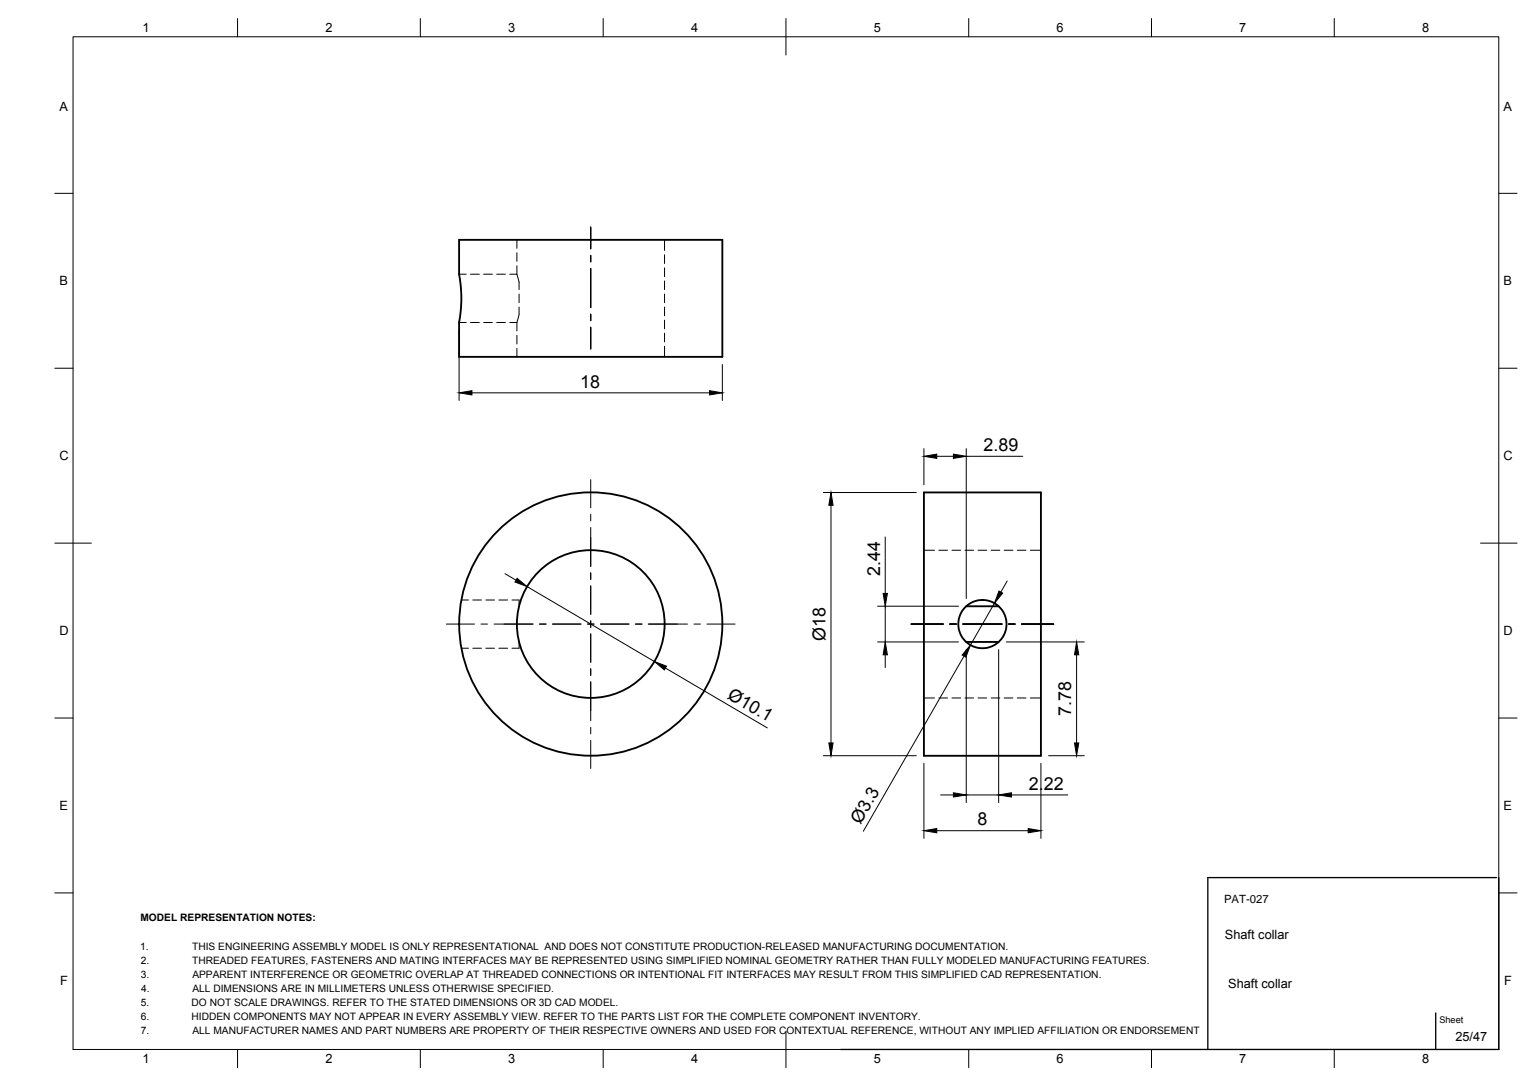
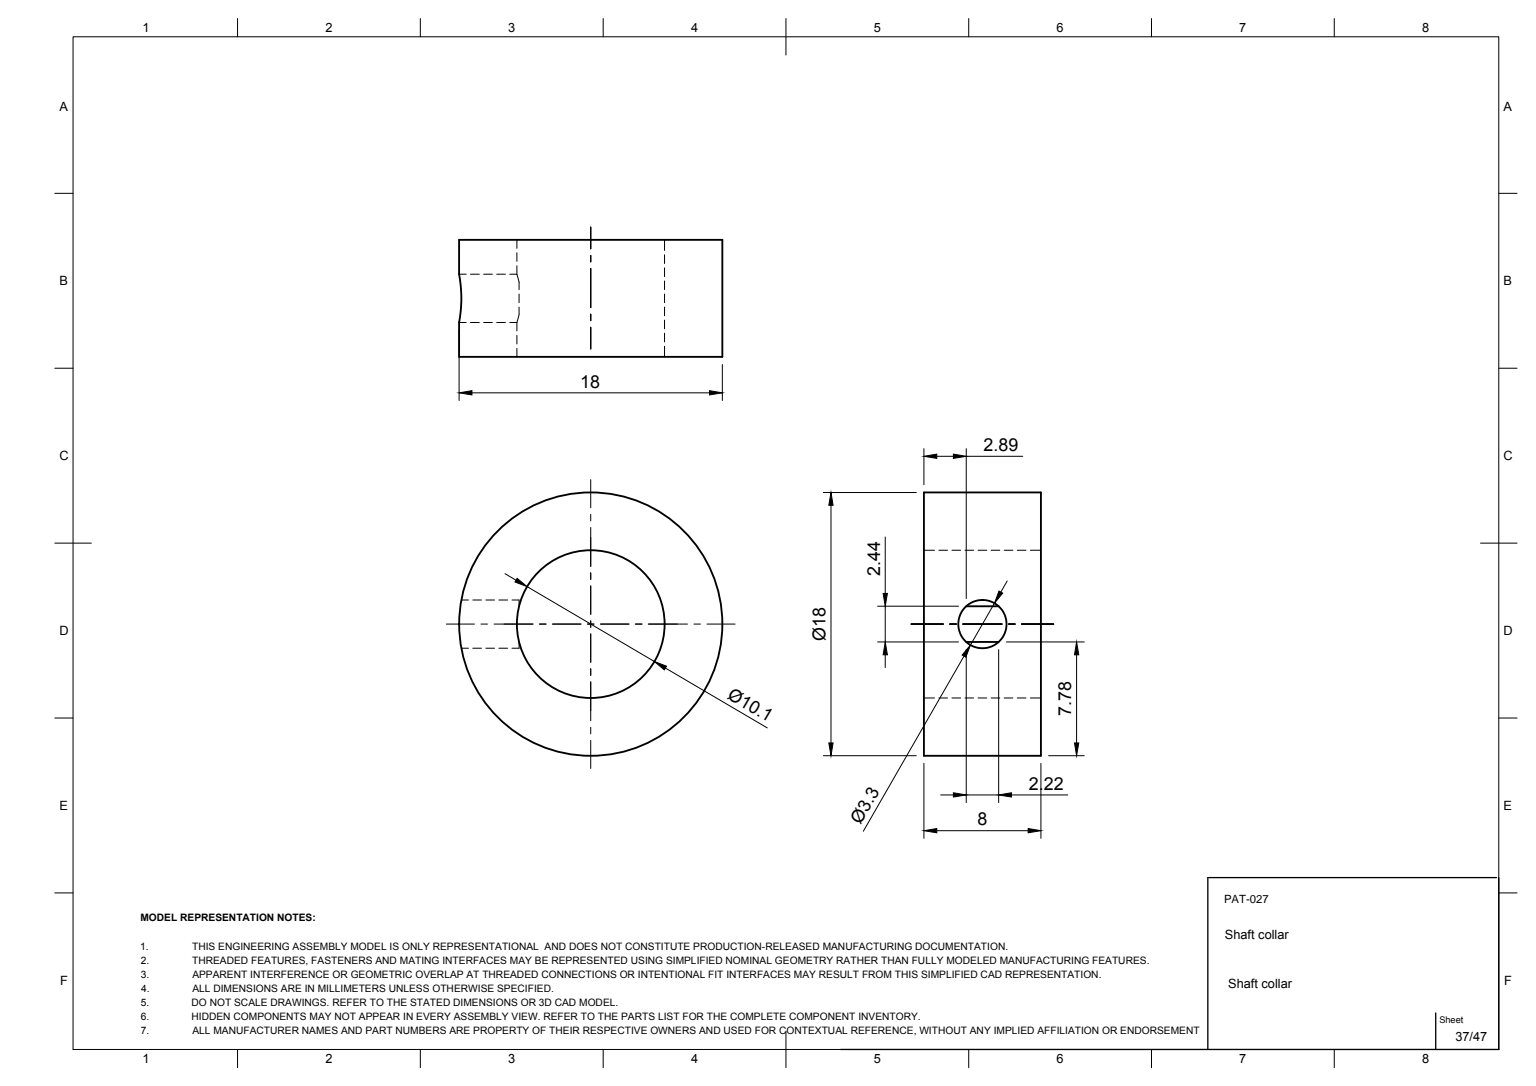
ISO-10303-21;
HEADER;
/* Generated by software containing ST-Developer
 * from STEP Tools, Inc. (www.steptools.com) 
 */

FILE_DESCRIPTION(
/* description */ ('Crank-driven oscillating fan base (mechanism only)'),

/* implementation_level */ '2;1');

FILE_NAME(
/* name */ 'Shaft collar.step',
/* time_stamp */ '2026-10-28T03:25:00-07:00',
/* author */ (''),
/* organization */ (''),
/* preprocessor_version */ 'ST-DEVELOPER v20.2',
/* originating_system */ 'Autodesk Translation Framework v15.17.0.0',
/* authorisation */ '');

FILE_SCHEMA (('AUTOMOTIVE_DESIGN { 1 0 10303 214 3 1 1 }'));
ENDSEC;

DATA;
#10=MECHANICAL_DESIGN_GEOMETRIC_PRESENTATION_REPRESENTATION('',(#462),#11916);
#342=B_SPLINE_CURVE_WITH_KNOTS('',3,(#10852,#10853,#10854,#10855,#10856,
#10857,#10858,#10859,#10860,#10861,#10862,#10863,#10864,#10865),
 .UNSPECIFIED.,.F.,.F.,(4,2,2,2,2,2,4),(0.618551524396293,0.626563103102765,
0.689203386094988,0.751843669087211,0.814483952079434,0.877124235071657,
0.88513581377813),.UNSPECIFIED.);
#343=B_SPLINE_CURVE_WITH_KNOTS('',3,(#10869,#10870,#10871,#10872,#10873,
#10874,#10875,#10876),.UNSPECIFIED.,.F.,.F.,(4,2,2,4),(0.250614556362404,
0.313254839354627,0.37589512234685,0.383906701053323),.UNSPECIFIED.);
#344=B_SPLINE_CURVE_WITH_KNOTS('',3,(#10880,#10881,#10882,#10883,#10884,
#10885,#10886,#10887,#10888,#10889,#10890,#10891,#10892,#10893,#10894,#10895,
#10896,#10897,#10898,#10899,#10900,#10901,#10902,#10903,#10904,#10905),
 .UNSPECIFIED.,.F.,.F.,(4,2,2,2,2,2,2,2,2,2,2,2,4),(0.,0.0623062782223143,
0.124612556444629,0.186916384615149,0.249220212785669,0.31152404095619,
0.37382786912671,0.436134147349024,0.498440425571339,0.560746703793653,
0.623052982015967,0.685356810186488,0.747660638357008),.UNSPECIFIED.);
#345=B_SPLINE_CURVE_WITH_KNOTS('',3,(#10906,#10907,#10908,#10909,#10910,
#10911,#10912,#10913,#10914,#10915),.UNSPECIFIED.,.F.,.F.,(4,2,2,2,4),(0.747660638357008,
0.809964466527528,0.872268294698049,0.934574572920363,0.996880851142677),
 .UNSPECIFIED.);
#346=B_SPLINE_CURVE_WITH_KNOTS('',3,(#10916,#10917,#10918,#10919,#10920,
#10921,#10922,#10923),.UNSPECIFIED.,.F.,.F.,(4,2,2,4),(0.117322411671485,
0.125333990377958,0.187974273370181,0.250614556362404),.UNSPECIFIED.);
#374=SHAPE_REPRESENTATION_RELATIONSHIP('SRR','None',#12100,#414);
#414=ADVANCED_BREP_SHAPE_REPRESENTATION('',(#509),#11891);
#462=STYLED_ITEM('',(#12375),#509);
#509=MANIFOLD_SOLID_BREP('Body1',#6093);
#626=FACE_BOUND('',#1559,.T.);
#627=FACE_BOUND('',#1561,.T.);
#628=FACE_BOUND('',#1563,.T.);
#629=FACE_BOUND('',#1565,.T.);
#782=PLANE('',#7013);
#783=PLANE('',#7017);
#784=PLANE('',#7024);
#785=PLANE('',#7025);
#1084=FACE_OUTER_BOUND('',#1555,.T.);
#1085=FACE_OUTER_BOUND('',#1556,.T.);
#1086=FACE_OUTER_BOUND('',#1557,.T.);
#1087=FACE_OUTER_BOUND('',#1558,.T.);
#1088=FACE_OUTER_BOUND('',#1560,.T.);
#1089=FACE_OUTER_BOUND('',#1562,.T.);
#1090=FACE_OUTER_BOUND('',#1564,.T.);
#1555=EDGE_LOOP('',(#4894,#4895));
#1556=EDGE_LOOP('',(#4896,#4897,#4898,#4899,#4900,#4901,#4902,#4903,#4904));
#1557=EDGE_LOOP('',(#4905,#4906));
#1558=EDGE_LOOP('',(#4907,#4908,#4909,#4910));
#1559=EDGE_LOOP('',(#4911,#4912,#4913,#4914,#4915));
#1560=EDGE_LOOP('',(#4916,#4917,#4918,#4919));
#1561=EDGE_LOOP('',(#4920,#4921));
#1562=EDGE_LOOP('',(#4922));
#1563=EDGE_LOOP('',(#4923));
#1564=EDGE_LOOP('',(#4924));
#1565=EDGE_LOOP('',(#4925));
#1956=LINE('',#10848,#2289);
#1957=LINE('',#10878,#2290);
#1958=LINE('',#10925,#2291);
#1959=LINE('',#10930,#2292);
#1960=LINE('',#10936,#2293);
#2289=VECTOR('',#8479,1.);
#2290=VECTOR('',#8486,0.165);
#2291=VECTOR('',#8489,1.);
#2292=VECTOR('',#8494,0.505);
#2293=VECTOR('',#8501,0.9);
#2693=CIRCLE('',#7014,0.165);
#2694=CIRCLE('',#7016,0.165);
#2695=CIRCLE('',#7019,0.505);
#2696=CIRCLE('',#7020,0.505);
#2697=CIRCLE('',#7022,0.9);
#2698=CIRCLE('',#7023,0.9);
#3114=VERTEX_POINT('',#10846);
#3115=VERTEX_POINT('',#10847);
#3116=VERTEX_POINT('',#10851);
#3117=VERTEX_POINT('',#10866);
#3118=VERTEX_POINT('',#10868);
#3119=VERTEX_POINT('',#10877);
#3120=VERTEX_POINT('',#10879);
#3121=VERTEX_POINT('',#10927);
#3122=VERTEX_POINT('',#10929);
#3123=VERTEX_POINT('',#10933);
#3124=VERTEX_POINT('',#10935);
#3742=EDGE_CURVE('',#3114,#3115,#1956,.T.);
#3743=EDGE_CURVE('',#3114,#3115,#2693,.T.);
#3744=EDGE_CURVE('',#3116,#3114,#342,.T.);
#3745=EDGE_CURVE('',#3117,#3116,#2694,.T.);
#3746=EDGE_CURVE('',#3118,#3117,#343,.T.);
#3747=EDGE_CURVE('',#3118,#3119,#1957,.T.);
#3748=EDGE_CURVE('',#3120,#3119,#344,.T.);
#3749=EDGE_CURVE('',#3119,#3120,#345,.T.);
#3750=EDGE_CURVE('',#3115,#3118,#346,.T.);
#3751=EDGE_CURVE('',#3117,#3116,#1958,.T.);
#3752=EDGE_CURVE('',#3121,#3121,#2695,.T.);
#3753=EDGE_CURVE('',#3121,#3122,#1959,.T.);
#3754=EDGE_CURVE('',#3122,#3122,#2696,.T.);
#3755=EDGE_CURVE('',#3123,#3123,#2697,.T.);
#3756=EDGE_CURVE('',#3123,#3124,#1960,.T.);
#3757=EDGE_CURVE('',#3124,#3124,#2698,.T.);
#4894=ORIENTED_EDGE('',*,*,#3742,.F.);
#4895=ORIENTED_EDGE('',*,*,#3743,.T.);
#4896=ORIENTED_EDGE('',*,*,#3744,.F.);
#4897=ORIENTED_EDGE('',*,*,#3745,.F.);
#4898=ORIENTED_EDGE('',*,*,#3746,.F.);
#4899=ORIENTED_EDGE('',*,*,#3747,.T.);
#4900=ORIENTED_EDGE('',*,*,#3748,.F.);
#4901=ORIENTED_EDGE('',*,*,#3749,.F.);
#4902=ORIENTED_EDGE('',*,*,#3747,.F.);
#4903=ORIENTED_EDGE('',*,*,#3750,.F.);
#4904=ORIENTED_EDGE('',*,*,#3743,.F.);
#4905=ORIENTED_EDGE('',*,*,#3751,.F.);
#4906=ORIENTED_EDGE('',*,*,#3745,.T.);
#4907=ORIENTED_EDGE('',*,*,#3752,.F.);
#4908=ORIENTED_EDGE('',*,*,#3753,.T.);
#4909=ORIENTED_EDGE('',*,*,#3754,.T.);
#4910=ORIENTED_EDGE('',*,*,#3753,.F.);
#4911=ORIENTED_EDGE('',*,*,#3750,.T.);
#4912=ORIENTED_EDGE('',*,*,#3746,.T.);
#4913=ORIENTED_EDGE('',*,*,#3751,.T.);
#4914=ORIENTED_EDGE('',*,*,#3744,.T.);
#4915=ORIENTED_EDGE('',*,*,#3742,.T.);
#4916=ORIENTED_EDGE('',*,*,#3755,.F.);
#4917=ORIENTED_EDGE('',*,*,#3756,.T.);
#4918=ORIENTED_EDGE('',*,*,#3757,.T.);
#4919=ORIENTED_EDGE('',*,*,#3756,.F.);
#4920=ORIENTED_EDGE('',*,*,#3748,.T.);
#4921=ORIENTED_EDGE('',*,*,#3749,.T.);
#4922=ORIENTED_EDGE('',*,*,#3755,.T.);
#4923=ORIENTED_EDGE('',*,*,#3752,.T.);
#4924=ORIENTED_EDGE('',*,*,#3757,.F.);
#4925=ORIENTED_EDGE('',*,*,#3754,.F.);
#5629=CYLINDRICAL_SURFACE('',#7015,0.165);
#5630=CYLINDRICAL_SURFACE('',#7018,0.505);
#5631=CYLINDRICAL_SURFACE('',#7021,0.9);
#5890=ADVANCED_FACE('',(#1084),#782,.T.);
#5891=ADVANCED_FACE('',(#1085),#5629,.F.);
#5892=ADVANCED_FACE('',(#1086),#783,.T.);
#5893=ADVANCED_FACE('',(#1087,#626),#5630,.F.);
#5894=ADVANCED_FACE('',(#1088,#627),#5631,.T.);
#5895=ADVANCED_FACE('',(#1089,#628),#784,.T.);
#5896=ADVANCED_FACE('',(#1090,#629),#785,.F.);
#6093=CLOSED_SHELL('',(#5890,#5891,#5892,#5893,#5894,#5895,#5896));
#7012=AXIS2_PLACEMENT_3D('',#10844,#8475,#8476);
#7013=AXIS2_PLACEMENT_3D('',#10845,#8477,#8478);
#7014=AXIS2_PLACEMENT_3D('',#10849,#8480,#8481);
#7015=AXIS2_PLACEMENT_3D('',#10850,#8482,#8483);
#7016=AXIS2_PLACEMENT_3D('',#10867,#8484,#8485);
#7017=AXIS2_PLACEMENT_3D('',#10924,#8487,#8488);
#7018=AXIS2_PLACEMENT_3D('',#10926,#8490,#8491);
#7019=AXIS2_PLACEMENT_3D('',#10928,#8492,#8493);
#7020=AXIS2_PLACEMENT_3D('',#10931,#8495,#8496);
#7021=AXIS2_PLACEMENT_3D('',#10932,#8497,#8498);
#7022=AXIS2_PLACEMENT_3D('',#10934,#8499,#8500);
#7023=AXIS2_PLACEMENT_3D('',#10937,#8502,#8503);
#7024=AXIS2_PLACEMENT_3D('',#10938,#8504,#8505);
#7025=AXIS2_PLACEMENT_3D('',#10939,#8506,#8507);
#8475=DIRECTION('axis',(0.,0.,1.));
#8476=DIRECTION('refdir',(1.,0.,0.));
#8477=DIRECTION('center_axis',(1.,0.,0.));
#8478=DIRECTION('ref_axis',(0.,0.,-1.));
#8479=DIRECTION('',(0.,0.,1.));
#8480=DIRECTION('center_axis',(1.,0.,0.));
#8481=DIRECTION('ref_axis',(0.,0.,-1.));
#8482=DIRECTION('center_axis',(1.,0.,0.));
#8483=DIRECTION('ref_axis',(0.,0.,-1.));
#8484=DIRECTION('center_axis',(1.,0.,0.));
#8485=DIRECTION('ref_axis',(0.,0.,-1.));
#8486=DIRECTION('',(1.,0.,0.));
#8487=DIRECTION('center_axis',(1.,0.,0.));
#8488=DIRECTION('ref_axis',(0.,0.,-1.));
#8489=DIRECTION('',(0.,0.,-1.));
#8490=DIRECTION('center_axis',(0.,0.,1.));
#8491=DIRECTION('ref_axis',(1.,0.,0.));
#8492=DIRECTION('center_axis',(0.,0.,-1.));
#8493=DIRECTION('ref_axis',(1.,0.,0.));
#8494=DIRECTION('',(0.,0.,-1.));
#8495=DIRECTION('center_axis',(0.,0.,-1.));
#8496=DIRECTION('ref_axis',(1.,0.,0.));
#8497=DIRECTION('center_axis',(0.,0.,1.));
#8498=DIRECTION('ref_axis',(1.,0.,0.));
#8499=DIRECTION('center_axis',(0.,0.,1.));
#8500=DIRECTION('ref_axis',(1.,0.,0.));
#8501=DIRECTION('',(0.,0.,-1.));
#8502=DIRECTION('center_axis',(0.,0.,1.));
#8503=DIRECTION('ref_axis',(1.,0.,0.));
#8504=DIRECTION('center_axis',(0.,0.,1.));
#8505=DIRECTION('ref_axis',(1.,0.,0.));
#8506=DIRECTION('center_axis',(0.,0.,1.));
#8507=DIRECTION('ref_axis',(1.,0.,0.));
#10844=CARTESIAN_POINT('',(0.,0.,0.));
#10845=CARTESIAN_POINT('Origin',(0.49,0.,1.4));
#10846=CARTESIAN_POINT('',(0.49,0.122167917228706,1.28909463493591));
#10847=CARTESIAN_POINT('',(0.49,0.122167917228706,1.51090536506409));
#10848=CARTESIAN_POINT('',(0.49,0.122167917228706,1.));
#10849=CARTESIAN_POINT('Origin',(0.49,0.,1.4));
#10850=CARTESIAN_POINT('Origin',(0.49,0.,1.4));
#10851=CARTESIAN_POINT('',(0.49,-0.122167917228706,1.28909463493591));
#10852=CARTESIAN_POINT('Ctrl Pts',(0.49,-0.122167917228706,1.28909463493591));
#10853=CARTESIAN_POINT('Ctrl Pts',(0.490448531679987,-0.120368913626296,
1.28711294069536));
#10854=CARTESIAN_POINT('Ctrl Pts',(0.490895245371685,-0.118534896565231,
1.28518965877367));
#10855=CARTESIAN_POINT('Ctrl Pts',(0.494795015531646,-0.102111993019358,
1.2687667552278));
#10856=CARTESIAN_POINT('Ctrl Pts',(0.498442514607594,-0.0836597150224318,
1.25609154388858));
#10857=CARTESIAN_POINT('Ctrl Pts',(0.50357781976106,-0.0430495960471595,
1.23920409039234));
#10858=CARTESIAN_POINT('Ctrl Pts',(0.505,-0.020880094330741,1.235));
#10859=CARTESIAN_POINT('Ctrl Pts',(0.505,0.020880094330741,1.235));
#10860=CARTESIAN_POINT('Ctrl Pts',(0.50357781976106,0.0430495960471595,
1.23920409039234));
#10861=CARTESIAN_POINT('Ctrl Pts',(0.498442514607594,0.0836597150224318,
1.25609154388858));
#10862=CARTESIAN_POINT('Ctrl Pts',(0.494795015531646,0.102111993019358,
1.2687667552278));
#10863=CARTESIAN_POINT('Ctrl Pts',(0.490895245371684,0.118534896565231,
1.28518965877367));
#10864=CARTESIAN_POINT('Ctrl Pts',(0.490448531679987,0.120368913626296,
1.28711294069536));
#10865=CARTESIAN_POINT('Ctrl Pts',(0.49,0.122167917228706,1.28909463493591));
#10866=CARTESIAN_POINT('',(0.49,-0.122167917228706,1.51090536506409));
#10867=CARTESIAN_POINT('Origin',(0.49,0.,1.4));
#10868=CARTESIAN_POINT('',(0.505,-1.70422299968729E-17,1.565));
#10869=CARTESIAN_POINT('Ctrl Pts',(0.505,-6.93889390390723E-18,1.565));
#10870=CARTESIAN_POINT('Ctrl Pts',(0.505,-0.020880094330741,1.565));
#10871=CARTESIAN_POINT('Ctrl Pts',(0.50357781976106,-0.0430495960471595,
1.56079590960766));
#10872=CARTESIAN_POINT('Ctrl Pts',(0.498442514607594,-0.0836597150224318,
1.54390845611142));
#10873=CARTESIAN_POINT('Ctrl Pts',(0.494795015531646,-0.102111993019358,
1.5312332447722));
#10874=CARTESIAN_POINT('Ctrl Pts',(0.490895245371684,-0.118534896565231,
1.51481034122633));
#10875=CARTESIAN_POINT('Ctrl Pts',(0.490448531679987,-0.120368913626296,
1.51288705930464));
#10876=CARTESIAN_POINT('Ctrl Pts',(0.49,-0.122167917228706,1.51090536506409));
#10877=CARTESIAN_POINT('',(0.9,-2.02066721859313E-17,1.565));
#10878=CARTESIAN_POINT('',(0.49,-2.02066721859313E-17,1.565));
#10879=CARTESIAN_POINT('',(0.884745726183518,0.165,1.4));
#10880=CARTESIAN_POINT('Ctrl Pts',(0.884745726183518,0.165,1.4));
#10881=CARTESIAN_POINT('Ctrl Pts',(0.884745726183518,0.165,1.37923124059256));
#10882=CARTESIAN_POINT('Ctrl Pts',(0.885552759505264,0.160839719007584,
1.35711110492666));
#10883=CARTESIAN_POINT('Ctrl Pts',(0.888448648150043,0.143986470216691,
1.31647293736623));
#10884=CARTESIAN_POINT('Ctrl Pts',(0.890493604851638,0.131295993814186,
1.29795075602263));
#10885=CARTESIAN_POINT('Ctrl Pts',(0.89431723432394,0.102049819008125,1.26870458121656));
#10886=CARTESIAN_POINT('Ctrl Pts',(0.896347088899543,0.0835273920906824,
1.25601365401642));
#10887=CARTESIAN_POINT('Ctrl Pts',(0.899208271860583,0.0428883760934127,
1.23916007816136));
#10888=CARTESIAN_POINT('Ctrl Pts',(0.9,0.0207679427235068,1.235));
#10889=CARTESIAN_POINT('Ctrl Pts',(0.9,-0.0207679427235068,1.235));
#10890=CARTESIAN_POINT('Ctrl Pts',(0.899208271860583,-0.0428883760934127,
1.23916007816136));
#10891=CARTESIAN_POINT('Ctrl Pts',(0.896347088899543,-0.0835273920906823,
1.25601365401642));
#10892=CARTESIAN_POINT('Ctrl Pts',(0.89431723432394,-0.102049819008125,
1.26870458121656));
#10893=CARTESIAN_POINT('Ctrl Pts',(0.890493604851638,-0.131295993814186,
1.29795075602263));
#10894=CARTESIAN_POINT('Ctrl Pts',(0.888448648150043,-0.143986470216691,
1.31647293736623));
#10895=CARTESIAN_POINT('Ctrl Pts',(0.885552759505264,-0.160839719007584,
1.35711110492666));
#10896=CARTESIAN_POINT('Ctrl Pts',(0.884745726183518,-0.165,1.37923124059256));
#10897=CARTESIAN_POINT('Ctrl Pts',(0.884745726183518,-0.165,1.42076875940744));
#10898=CARTESIAN_POINT('Ctrl Pts',(0.885552759505264,-0.160839719007584,
1.44288889507334));
#10899=CARTESIAN_POINT('Ctrl Pts',(0.888448648150043,-0.14398647021669,
1.48352706263377));
#10900=CARTESIAN_POINT('Ctrl Pts',(0.890493604851638,-0.131295993814186,
1.50204924397737));
#10901=CARTESIAN_POINT('Ctrl Pts',(0.89431723432394,-0.102049819008125,
1.53129541878344));
#10902=CARTESIAN_POINT('Ctrl Pts',(0.896347088899543,-0.0835273920906824,
1.54398634598358));
#10903=CARTESIAN_POINT('Ctrl Pts',(0.899208271860583,-0.0428883760934128,
1.56083992183864));
#10904=CARTESIAN_POINT('Ctrl Pts',(0.9,-0.0207679427235068,1.565));
#10905=CARTESIAN_POINT('Ctrl Pts',(0.9,-6.93889390390723E-18,1.565));
#10906=CARTESIAN_POINT('Ctrl Pts',(0.9,-3.46944695195361E-17,1.565));
#10907=CARTESIAN_POINT('Ctrl Pts',(0.9,0.0207679427235068,1.565));
#10908=CARTESIAN_POINT('Ctrl Pts',(0.899208271860583,0.0428883760934127,
1.56083992183864));
#10909=CARTESIAN_POINT('Ctrl Pts',(0.896347088899543,0.0835273920906824,
1.54398634598358));
#10910=CARTESIAN_POINT('Ctrl Pts',(0.89431723432394,0.102049819008125,1.53129541878344));
#10911=CARTESIAN_POINT('Ctrl Pts',(0.890493604851638,0.131295993814186,
1.50204924397737));
#10912=CARTESIAN_POINT('Ctrl Pts',(0.888448648150043,0.143986470216691,
1.48352706263377));
#10913=CARTESIAN_POINT('Ctrl Pts',(0.885552759505264,0.160839719007584,
1.44288889507334));
#10914=CARTESIAN_POINT('Ctrl Pts',(0.884745726183518,0.165,1.42076875940744));
#10915=CARTESIAN_POINT('Ctrl Pts',(0.884745726183518,0.165,1.4));
#10916=CARTESIAN_POINT('Ctrl Pts',(0.49,0.122167917228706,1.51090536506409));
#10917=CARTESIAN_POINT('Ctrl Pts',(0.490448531679987,0.120368913626296,
1.51288705930464));
#10918=CARTESIAN_POINT('Ctrl Pts',(0.490895245371685,0.118534896565231,
1.51481034122633));
#10919=CARTESIAN_POINT('Ctrl Pts',(0.494795015531646,0.102111993019358,
1.5312332447722));
#10920=CARTESIAN_POINT('Ctrl Pts',(0.498442514607594,0.0836597150224318,
1.54390845611142));
#10921=CARTESIAN_POINT('Ctrl Pts',(0.50357781976106,0.0430495960471594,
1.56079590960766));
#10922=CARTESIAN_POINT('Ctrl Pts',(0.505,0.020880094330741,1.565));
#10923=CARTESIAN_POINT('Ctrl Pts',(0.505,0.,1.565));
#10924=CARTESIAN_POINT('Origin',(0.49,0.,1.4));
#10925=CARTESIAN_POINT('',(0.49,-0.122167917228706,1.));
#10926=CARTESIAN_POINT('Origin',(0.,0.,1.));
#10927=CARTESIAN_POINT('',(-0.505,-6.18446633569413E-17,1.8));
#10928=CARTESIAN_POINT('Origin',(0.,0.,1.8));
#10929=CARTESIAN_POINT('',(-0.505,-6.18446633569413E-17,1.));
#10930=CARTESIAN_POINT('',(-0.505,-6.18446633569413E-17,1.));
#10931=CARTESIAN_POINT('Origin',(0.,0.,1.));
#10932=CARTESIAN_POINT('Origin',(0.,0.,1.));
#10933=CARTESIAN_POINT('',(-0.9,-1.10218211923262E-16,1.8));
#10934=CARTESIAN_POINT('Origin',(0.,0.,1.8));
#10935=CARTESIAN_POINT('',(-0.9,-1.10218211923262E-16,1.));
#10936=CARTESIAN_POINT('',(-0.9,-1.10218211923262E-16,1.));
#10937=CARTESIAN_POINT('Origin',(0.,0.,1.));
#10938=CARTESIAN_POINT('Origin',(0.,0.,1.8));
#10939=CARTESIAN_POINT('Origin',(0.,0.,1.));
#11844=UNCERTAINTY_MEASURE_WITH_UNIT(LENGTH_MEASURE(0.001),#11917,
'DISTANCE_ACCURACY_VALUE',
'Maximum model space distance between geometric entities at asserted c
onnectivities');
#11869=UNCERTAINTY_MEASURE_WITH_UNIT(LENGTH_MEASURE(0.001),#11917,
'DISTANCE_ACCURACY_VALUE',
'Maximum model space distance between geometric entities at asserted c
onnectivities');
#11891=(
GEOMETRIC_REPRESENTATION_CONTEXT(3)
GLOBAL_UNCERTAINTY_ASSIGNED_CONTEXT((#11844))
GLOBAL_UNIT_ASSIGNED_CONTEXT((#11917,#11919,#11920))
REPRESENTATION_CONTEXT('','3D')
);
#11916=(
GEOMETRIC_REPRESENTATION_CONTEXT(3)
GLOBAL_UNCERTAINTY_ASSIGNED_CONTEXT((#11869))
GLOBAL_UNIT_ASSIGNED_CONTEXT((#11917,#11919,#11920))
REPRESENTATION_CONTEXT('','3D')
);
#11917=(
LENGTH_UNIT()
NAMED_UNIT(*)
SI_UNIT(.CENTI.,.METRE.)
);
#11919=(
NAMED_UNIT(*)
PLANE_ANGLE_UNIT()
SI_UNIT($,.RADIAN.)
);
#11920=(
NAMED_UNIT(*)
SI_UNIT($,.STERADIAN.)
SOLID_ANGLE_UNIT()
);
#11942=SHAPE_DEFINITION_REPRESENTATION(#11993,#12100);
#11993=PRODUCT_DEFINITION_SHAPE('',$,#12147);
#12100=SHAPE_REPRESENTATION('',(#7012),#11891);
#12125=PRODUCT_DEFINITION_CONTEXT('part definition',#12265,'design');
#12147=PRODUCT_DEFINITION('Shaft collar','Shaft collar',#12193,#12125);
#12193=PRODUCT_DEFINITION_FORMATION('',$,#12288);
#12265=APPLICATION_CONTEXT(
'Core Data for Automotive Mechanical Design Process');
#12266=PRODUCT_CONTEXT('part definition',#12265,'mechanical');
#12288=PRODUCT('Shaft collar','Shaft collar','Shaft collar',(#12266));
#12369=COLOUR_RGB('Grey',0.48,0.52,0.57);
#12370=FILL_AREA_STYLE_COLOUR('',#12369);
#12371=FILL_AREA_STYLE('',(#12370));
#12372=SURFACE_STYLE_FILL_AREA(#12371);
#12373=SURFACE_SIDE_STYLE('',(#12372));
#12374=SURFACE_STYLE_USAGE(.BOTH.,#12373);
#12375=PRESENTATION_STYLE_ASSIGNMENT((#12374));
ENDSEC;
END-ISO-10303-21;
